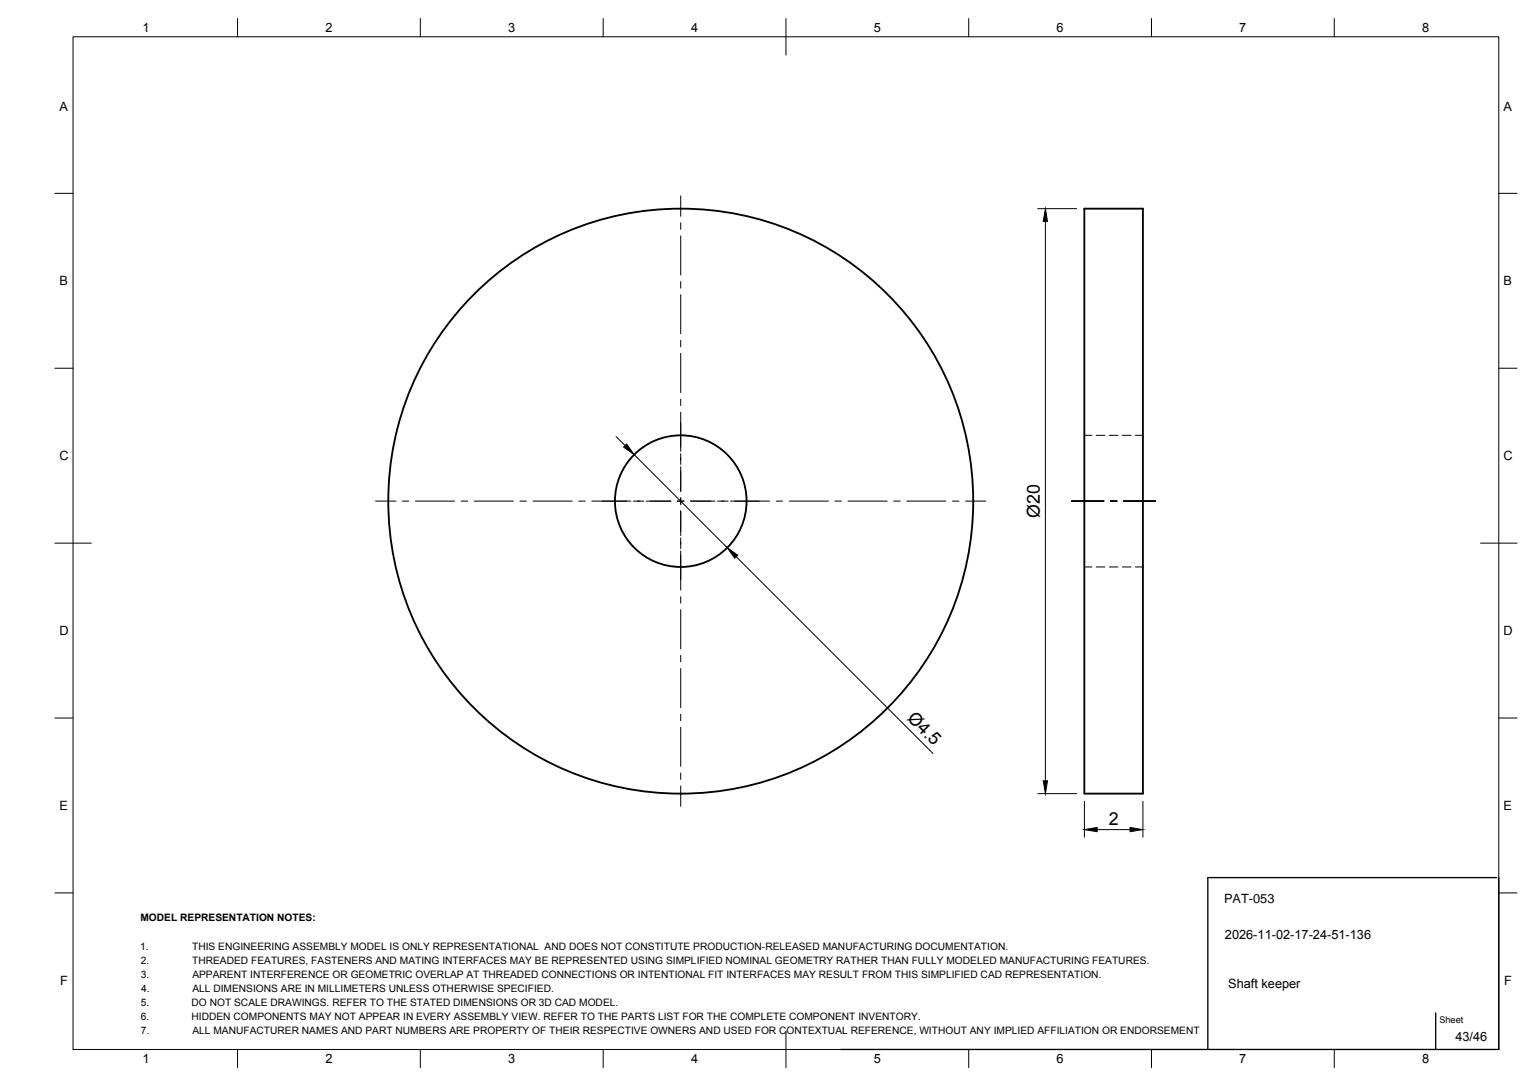
ISO-10303-21;
HEADER;
/* Generated by software containing ST-Developer
 * from STEP Tools, Inc. (www.steptools.com) 
 */

FILE_DESCRIPTION(
/* description */ ('Hand-operated arbor press'),
/* implementation_level */ '2;1');

FILE_NAME(
/* name */ 'Shaft keeper.step',
/* time_stamp */ '2026-10-28T03:25:25-07:00',
/* author */ (''),
/* organization */ (''),
/* preprocessor_version */ 'ST-DEVELOPER v20.2',
/* originating_system */ 'Autodesk Translation Framework v15.17.0.0',
/* authorisation */ '');

FILE_SCHEMA (('AUTOMOTIVE_DESIGN { 1 0 10303 214 3 1 1 }'));
ENDSEC;

DATA;
#10=MECHANICAL_DESIGN_GEOMETRIC_PRESENTATION_REPRESENTATION('',(#628),#32751);
#537=SHAPE_REPRESENTATION_RELATIONSHIP('SRR','None',#32969,#579);
#579=ADVANCED_BREP_SHAPE_REPRESENTATION('',(#675),#32743);
#628=STYLED_ITEM('',(#33242),#675);
#675=MANIFOLD_SOLID_BREP('Body1',#12527);
#836=FACE_BOUND('',#2676,.T.);
#837=FACE_BOUND('',#2678,.T.);
#1237=PLANE('',#13912);
#1238=PLANE('',#13913);
#1836=FACE_OUTER_BOUND('',#2673,.T.);
#1837=FACE_OUTER_BOUND('',#2674,.T.);
#1838=FACE_OUTER_BOUND('',#2675,.T.);
#1839=FACE_OUTER_BOUND('',#2677,.T.);
#2673=EDGE_LOOP('',(#10956,#10957,#10958,#10959));
#2674=EDGE_LOOP('',(#10960,#10961,#10962,#10963));
#2675=EDGE_LOOP('',(#10964));
#2676=EDGE_LOOP('',(#10965));
#2677=EDGE_LOOP('',(#10966));
#2678=EDGE_LOOP('',(#10967));
#3808=LINE('',#20796,#4979);
#3809=LINE('',#20802,#4980);
#4979=VECTOR('',#16957,0.225);
#4980=VECTOR('',#16964,1.);
#5480=CIRCLE('',#13907,0.225);
#5481=CIRCLE('',#13908,0.225);
#5482=CIRCLE('',#13910,1.);
#5483=CIRCLE('',#13911,1.);
#6439=VERTEX_POINT('',#20793);
#6440=VERTEX_POINT('',#20795);
#6441=VERTEX_POINT('',#20799);
#6442=VERTEX_POINT('',#20801);
#7981=EDGE_CURVE('',#6439,#6439,#5480,.T.);
#7982=EDGE_CURVE('',#6439,#6440,#3808,.T.);
#7983=EDGE_CURVE('',#6440,#6440,#5481,.T.);
#7984=EDGE_CURVE('',#6441,#6441,#5482,.T.);
#7985=EDGE_CURVE('',#6441,#6442,#3809,.T.);
#7986=EDGE_CURVE('',#6442,#6442,#5483,.T.);
#10956=ORIENTED_EDGE('',*,*,#7981,.F.);
#10957=ORIENTED_EDGE('',*,*,#7982,.T.);
#10958=ORIENTED_EDGE('',*,*,#7983,.T.);
#10959=ORIENTED_EDGE('',*,*,#7982,.F.);
#10960=ORIENTED_EDGE('',*,*,#7984,.F.);
#10961=ORIENTED_EDGE('',*,*,#7985,.T.);
#10962=ORIENTED_EDGE('',*,*,#7986,.T.);
#10963=ORIENTED_EDGE('',*,*,#7985,.F.);
#10964=ORIENTED_EDGE('',*,*,#7984,.T.);
#10965=ORIENTED_EDGE('',*,*,#7981,.T.);
#10966=ORIENTED_EDGE('',*,*,#7986,.F.);
#10967=ORIENTED_EDGE('',*,*,#7983,.F.);
#11768=CYLINDRICAL_SURFACE('',#13906,0.225);
#11769=CYLINDRICAL_SURFACE('',#13909,1.);
#12345=ADVANCED_FACE('',(#1836),#11768,.F.);
#12346=ADVANCED_FACE('',(#1837),#11769,.T.);
#12347=ADVANCED_FACE('',(#1838,#836),#1237,.T.);
#12348=ADVANCED_FACE('',(#1839,#837),#1238,.F.);
#12527=CLOSED_SHELL('',(#12345,#12346,#12347,#12348));
#13905=AXIS2_PLACEMENT_3D('',#20791,#16951,#16952);
#13906=AXIS2_PLACEMENT_3D('',#20792,#16953,#16954);
#13907=AXIS2_PLACEMENT_3D('',#20794,#16955,#16956);
#13908=AXIS2_PLACEMENT_3D('',#20797,#16958,#16959);
#13909=AXIS2_PLACEMENT_3D('',#20798,#16960,#16961);
#13910=AXIS2_PLACEMENT_3D('',#20800,#16962,#16963);
#13911=AXIS2_PLACEMENT_3D('',#20803,#16965,#16966);
#13912=AXIS2_PLACEMENT_3D('',#20804,#16967,#16968);
#13913=AXIS2_PLACEMENT_3D('',#20805,#16969,#16970);
#16951=DIRECTION('axis',(0.,0.,1.));
#16952=DIRECTION('refdir',(1.,0.,0.));
#16953=DIRECTION('center_axis',(0.,1.,0.));
#16954=DIRECTION('ref_axis',(1.,0.,0.));
#16955=DIRECTION('center_axis',(0.,-1.,0.));
#16956=DIRECTION('ref_axis',(1.,0.,0.));
#16957=DIRECTION('',(0.,-1.,0.));
#16958=DIRECTION('center_axis',(0.,-1.,0.));
#16959=DIRECTION('ref_axis',(1.,0.,0.));
#16960=DIRECTION('center_axis',(0.,1.,0.));
#16961=DIRECTION('ref_axis',(1.,0.,0.));
#16962=DIRECTION('center_axis',(0.,1.,0.));
#16963=DIRECTION('ref_axis',(1.,0.,0.));
#16964=DIRECTION('',(0.,-1.,0.));
#16965=DIRECTION('center_axis',(0.,1.,0.));
#16966=DIRECTION('ref_axis',(1.,0.,0.));
#16967=DIRECTION('center_axis',(0.,1.,0.));
#16968=DIRECTION('ref_axis',(1.,0.,0.));
#16969=DIRECTION('center_axis',(0.,1.,0.));
#16970=DIRECTION('ref_axis',(1.,0.,0.));
#20791=CARTESIAN_POINT('',(0.,0.,0.));
#20792=CARTESIAN_POINT('Origin',(-3.25,-5.7,20.));
#20793=CARTESIAN_POINT('',(-3.475,-5.5,20.));
#20794=CARTESIAN_POINT('Origin',(-3.25,-5.5,20.));
#20795=CARTESIAN_POINT('',(-3.475,-5.7,20.));
#20796=CARTESIAN_POINT('',(-3.475,-5.7,20.));
#20797=CARTESIAN_POINT('Origin',(-3.25,-5.7,20.));
#20798=CARTESIAN_POINT('Origin',(-3.25,-5.7,20.));
#20799=CARTESIAN_POINT('',(-4.25,-5.5,20.));
#20800=CARTESIAN_POINT('Origin',(-3.25,-5.5,20.));
#20801=CARTESIAN_POINT('',(-4.25,-5.7,20.));
#20802=CARTESIAN_POINT('',(-4.25,-5.7,20.));
#20803=CARTESIAN_POINT('Origin',(-3.25,-5.7,20.));
#20804=CARTESIAN_POINT('Origin',(-3.25,-5.5,20.));
#20805=CARTESIAN_POINT('Origin',(-3.25,-5.7,20.));
#32694=UNCERTAINTY_MEASURE_WITH_UNIT(LENGTH_MEASURE(0.001),#32752,
'DISTANCE_ACCURACY_VALUE',
'Maximum model space distance between geometric entities at asserted c
onnectivities');
#32702=UNCERTAINTY_MEASURE_WITH_UNIT(LENGTH_MEASURE(0.001),#32752,
'DISTANCE_ACCURACY_VALUE',
'Maximum model space distance between geometric entities at asserted c
onnectivities');
#32743=(
GEOMETRIC_REPRESENTATION_CONTEXT(3)
GLOBAL_UNCERTAINTY_ASSIGNED_CONTEXT((#32694))
GLOBAL_UNIT_ASSIGNED_CONTEXT((#32752,#32754,#32755))
REPRESENTATION_CONTEXT('','3D')
);
#32751=(
GEOMETRIC_REPRESENTATION_CONTEXT(3)
GLOBAL_UNCERTAINTY_ASSIGNED_CONTEXT((#32702))
GLOBAL_UNIT_ASSIGNED_CONTEXT((#32752,#32754,#32755))
REPRESENTATION_CONTEXT('','3D')
);
#32752=(
LENGTH_UNIT()
NAMED_UNIT(*)
SI_UNIT(.CENTI.,.METRE.)
);
#32754=(
NAMED_UNIT(*)
PLANE_ANGLE_UNIT()
SI_UNIT($,.RADIAN.)
);
#32755=(
NAMED_UNIT(*)
SI_UNIT($,.STERADIAN.)
SOLID_ANGLE_UNIT()
);
#32796=SHAPE_DEFINITION_REPRESENTATION(#32853,#32969);
#32853=PRODUCT_DEFINITION_SHAPE('',$,#33018);
#32969=SHAPE_REPRESENTATION('',(#13905),#32743);
#32977=PRODUCT_DEFINITION_CONTEXT('part definition',#33123,'design');
#33018=PRODUCT_DEFINITION('Shaft keeper','Shaft keeper',#33066,#32977);
#33066=PRODUCT_DEFINITION_FORMATION('',$,#33165);
#33123=APPLICATION_CONTEXT(
'Core Data for Automotive Mechanical Design Process');
#33124=PRODUCT_CONTEXT('part definition',#33123,'mechanical');
#33165=PRODUCT('Shaft keeper','Shaft keeper','Shaft keeper',(#33124));
#33236=COLOUR_RGB('Grey',0.48,0.52,0.57);
#33237=FILL_AREA_STYLE_COLOUR('',#33236);
#33238=FILL_AREA_STYLE('',(#33237));
#33239=SURFACE_STYLE_FILL_AREA(#33238);
#33240=SURFACE_SIDE_STYLE('',(#33239));
#33241=SURFACE_STYLE_USAGE(.BOTH.,#33240);
#33242=PRESENTATION_STYLE_ASSIGNMENT((#33241));
ENDSEC;
END-ISO-10303-21;
